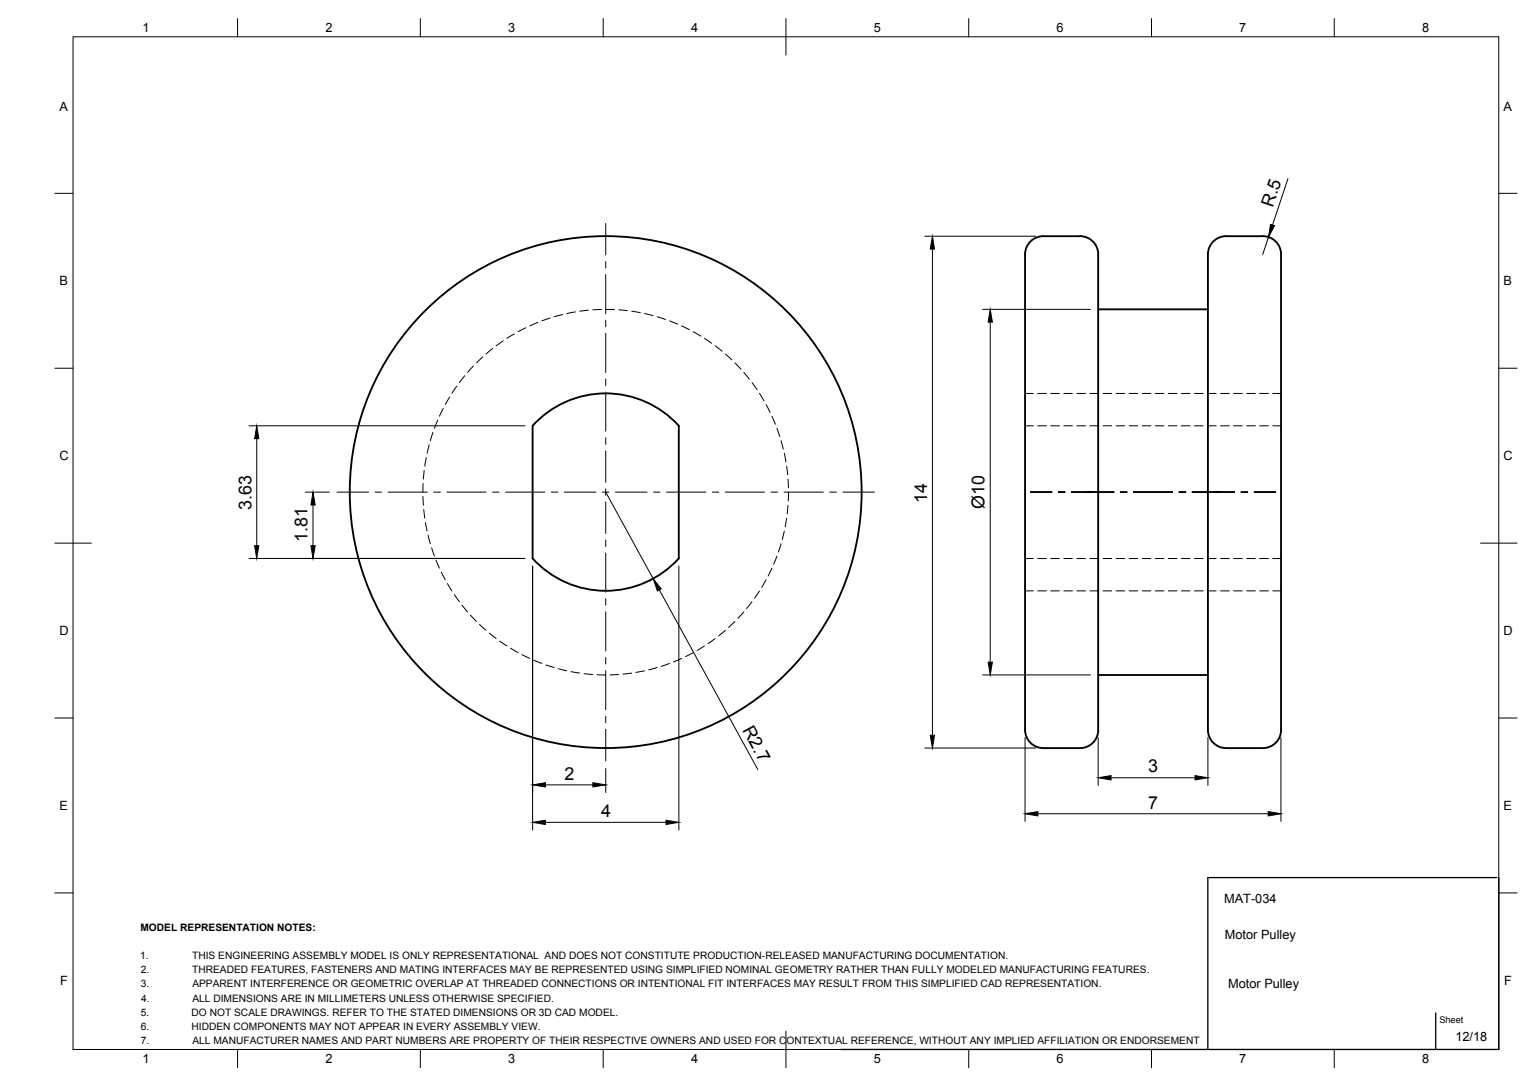
ISO-10303-21;
HEADER;
/* Generated by software containing ST-Developer
 * from STEP Tools, Inc. (www.steptools.com) 
 */

FILE_DESCRIPTION(
/* description */ ('STEP AP214'),
/* implementation_level */ '2;1');

FILE_NAME(
/* name */ 'Motor Pulley.step',
/* time_stamp */ '2026-11-14T09:24:36-08:00',
/* author */ (''),
/* organization */ (''),
/* preprocessor_version */ 'ST-DEVELOPER v20.2',
/* originating_system */ 'Autodesk Translation Framework v15.17.0.0',
/* authorisation */ '');

FILE_SCHEMA (('AUTOMOTIVE_DESIGN { 1 0 10303 214 3 1 1 }'));
ENDSEC;

DATA;
#10=MECHANICAL_DESIGN_GEOMETRIC_PRESENTATION_REPRESENTATION('',(#208),#18867);
#146=TOROIDAL_SURFACE('',#11512,6.5,0.5);
#147=TOROIDAL_SURFACE('',#11516,6.5,0.5);
#148=TOROIDAL_SURFACE('',#11521,6.5,0.5);
#149=TOROIDAL_SURFACE('',#11525,6.5,0.5);
#176=SHAPE_REPRESENTATION_RELATIONSHIP('SRR','None',#18940,#192);
#192=ADVANCED_BREP_SHAPE_REPRESENTATION('',(#232),#18856);
#208=STYLED_ITEM('',(#19027),#232);
#232=MANIFOLD_SOLID_BREP('Body1',#10963);
#319=FACE_BOUND('',#1599,.T.);
#320=FACE_BOUND('',#1601,.T.);
#321=FACE_BOUND('',#1603,.T.);
#322=FACE_BOUND('',#1605,.T.);
#513=PLANE('',#11535);
#514=PLANE('',#11536);
#515=PLANE('',#11537);
#516=PLANE('',#11540);
#517=PLANE('',#11543);
#518=PLANE('',#11545);
#927=FACE_OUTER_BOUND('',#1591,.T.);
#928=FACE_OUTER_BOUND('',#1592,.T.);
#929=FACE_OUTER_BOUND('',#1593,.T.);
#930=FACE_OUTER_BOUND('',#1594,.T.);
#931=FACE_OUTER_BOUND('',#1595,.T.);
#932=FACE_OUTER_BOUND('',#1596,.T.);
#933=FACE_OUTER_BOUND('',#1597,.T.);
#934=FACE_OUTER_BOUND('',#1598,.T.);
#935=FACE_OUTER_BOUND('',#1600,.T.);
#936=FACE_OUTER_BOUND('',#1602,.T.);
#937=FACE_OUTER_BOUND('',#1604,.T.);
#938=FACE_OUTER_BOUND('',#1606,.T.);
#939=FACE_OUTER_BOUND('',#1607,.T.);
#940=FACE_OUTER_BOUND('',#1608,.T.);
#941=FACE_OUTER_BOUND('',#1609,.T.);
#1591=EDGE_LOOP('',(#8120,#8121,#8122,#8123));
#1592=EDGE_LOOP('',(#8124,#8125,#8126,#8127,#8128));
#1593=EDGE_LOOP('',(#8129,#8130,#8131,#8132));
#1594=EDGE_LOOP('',(#8133,#8134,#8135,#8136,#8137));
#1595=EDGE_LOOP('',(#8138,#8139,#8140,#8141,#8142));
#1596=EDGE_LOOP('',(#8143,#8144,#8145,#8146));
#1597=EDGE_LOOP('',(#8147,#8148,#8149,#8150,#8151));
#1598=EDGE_LOOP('',(#8152));
#1599=EDGE_LOOP('',(#8153));
#1600=EDGE_LOOP('',(#8154));
#1601=EDGE_LOOP('',(#8155));
#1602=EDGE_LOOP('',(#8156));
#1603=EDGE_LOOP('',(#8157,#8158,#8159,#8160));
#1604=EDGE_LOOP('',(#8161));
#1605=EDGE_LOOP('',(#8162,#8163,#8164,#8165));
#1606=EDGE_LOOP('',(#8166,#8167,#8168,#8169));
#1607=EDGE_LOOP('',(#8170,#8171,#8172,#8173));
#1608=EDGE_LOOP('',(#8174,#8175,#8176,#8177));
#1609=EDGE_LOOP('',(#8178,#8179,#8180,#8181));
#2409=LINE('',#16685,#3423);
#2410=LINE('',#16690,#3424);
#2411=LINE('',#16693,#3425);
#2412=LINE('',#16701,#3426);
#2413=LINE('',#16704,#3427);
#2414=LINE('',#16710,#3428);
#2415=LINE('',#16713,#3429);
#2416=LINE('',#16715,#3430);
#2417=LINE('',#16716,#3431);
#2418=LINE('',#16718,#3432);
#2419=LINE('',#16720,#3433);
#3423=VECTOR('',#13409,7.);
#3424=VECTOR('',#13414,5.);
#3425=VECTOR('',#13419,7.);
#3426=VECTOR('',#13428,1000.);
#3427=VECTOR('',#13431,1000.);
#3428=VECTOR('',#13436,1000.);
#3429=VECTOR('',#13439,1000.);
#3430=VECTOR('',#13442,1000.);
#3431=VECTOR('',#13443,1000.);
#3432=VECTOR('',#13446,1000.);
#3433=VECTOR('',#13449,1000.);
#4215=CIRCLE('',#11513,7.);
#4216=CIRCLE('',#11514,0.5);
#4217=CIRCLE('',#11515,6.5);
#4218=CIRCLE('',#11517,7.);
#4219=CIRCLE('',#11518,7.);
#4220=CIRCLE('',#11519,0.5);
#4221=CIRCLE('',#11520,6.5);
#4222=CIRCLE('',#11522,7.);
#4223=CIRCLE('',#11523,0.5);
#4224=CIRCLE('',#11524,6.5);
#4225=CIRCLE('',#11526,7.);
#4226=CIRCLE('',#11527,7.);
#4227=CIRCLE('',#11528,0.5);
#4228=CIRCLE('',#11529,6.5);
#4229=CIRCLE('',#11532,5.);
#4230=CIRCLE('',#11533,5.);
#4231=CIRCLE('',#11538,2.7);
#4232=CIRCLE('',#11539,2.7);
#4233=CIRCLE('',#11541,2.7);
#4234=CIRCLE('',#11542,2.7);
#4910=VERTEX_POINT('',#16657);
#4911=VERTEX_POINT('',#16659);
#4912=VERTEX_POINT('',#16663);
#4913=VERTEX_POINT('',#16664);
#4914=VERTEX_POINT('',#16667);
#4915=VERTEX_POINT('',#16671);
#4916=VERTEX_POINT('',#16673);
#4917=VERTEX_POINT('',#16677);
#4918=VERTEX_POINT('',#16678);
#4919=VERTEX_POINT('',#16681);
#4920=VERTEX_POINT('',#16687);
#4921=VERTEX_POINT('',#16689);
#4922=VERTEX_POINT('',#16697);
#4923=VERTEX_POINT('',#16698);
#4924=VERTEX_POINT('',#16700);
#4925=VERTEX_POINT('',#16702);
#4926=VERTEX_POINT('',#16706);
#4927=VERTEX_POINT('',#16707);
#4928=VERTEX_POINT('',#16709);
#4929=VERTEX_POINT('',#16711);
#6093=EDGE_CURVE('',#4910,#4910,#4215,.T.);
#6094=EDGE_CURVE('',#4910,#4911,#4216,.T.);
#6095=EDGE_CURVE('',#4911,#4911,#4217,.T.);
#6096=EDGE_CURVE('',#4912,#4913,#4218,.T.);
#6097=EDGE_CURVE('',#4913,#4912,#4219,.T.);
#6098=EDGE_CURVE('',#4913,#4914,#4220,.T.);
#6099=EDGE_CURVE('',#4914,#4914,#4221,.T.);
#6100=EDGE_CURVE('',#4915,#4915,#4222,.T.);
#6101=EDGE_CURVE('',#4915,#4916,#4223,.T.);
#6102=EDGE_CURVE('',#4916,#4916,#4224,.T.);
#6103=EDGE_CURVE('',#4917,#4918,#4225,.T.);
#6104=EDGE_CURVE('',#4918,#4917,#4226,.T.);
#6105=EDGE_CURVE('',#4918,#4919,#4227,.T.);
#6106=EDGE_CURVE('',#4919,#4919,#4228,.T.);
#6107=EDGE_CURVE('',#4912,#4910,#2409,.T.);
#6108=EDGE_CURVE('',#4920,#4920,#4229,.T.);
#6109=EDGE_CURVE('',#4920,#4921,#2410,.T.);
#6110=EDGE_CURVE('',#4921,#4921,#4230,.T.);
#6111=EDGE_CURVE('',#4917,#4915,#2411,.T.);
#6112=EDGE_CURVE('',#4922,#4923,#4231,.T.);
#6113=EDGE_CURVE('',#4923,#4924,#2412,.T.);
#6114=EDGE_CURVE('',#4924,#4925,#4232,.T.);
#6115=EDGE_CURVE('',#4922,#4925,#2413,.T.);
#6116=EDGE_CURVE('',#4926,#4927,#4233,.T.);
#6117=EDGE_CURVE('',#4928,#4926,#2414,.T.);
#6118=EDGE_CURVE('',#4929,#4928,#4234,.T.);
#6119=EDGE_CURVE('',#4929,#4927,#2415,.T.);
#6120=EDGE_CURVE('',#4923,#4928,#2416,.T.);
#6121=EDGE_CURVE('',#4924,#4926,#2417,.T.);
#6122=EDGE_CURVE('',#4922,#4929,#2418,.T.);
#6123=EDGE_CURVE('',#4925,#4927,#2419,.T.);
#8120=ORIENTED_EDGE('',*,*,#6093,.F.);
#8121=ORIENTED_EDGE('',*,*,#6094,.T.);
#8122=ORIENTED_EDGE('',*,*,#6095,.F.);
#8123=ORIENTED_EDGE('',*,*,#6094,.F.);
#8124=ORIENTED_EDGE('',*,*,#6096,.F.);
#8125=ORIENTED_EDGE('',*,*,#6097,.F.);
#8126=ORIENTED_EDGE('',*,*,#6098,.T.);
#8127=ORIENTED_EDGE('',*,*,#6099,.F.);
#8128=ORIENTED_EDGE('',*,*,#6098,.F.);
#8129=ORIENTED_EDGE('',*,*,#6100,.F.);
#8130=ORIENTED_EDGE('',*,*,#6101,.T.);
#8131=ORIENTED_EDGE('',*,*,#6102,.F.);
#8132=ORIENTED_EDGE('',*,*,#6101,.F.);
#8133=ORIENTED_EDGE('',*,*,#6103,.F.);
#8134=ORIENTED_EDGE('',*,*,#6104,.F.);
#8135=ORIENTED_EDGE('',*,*,#6105,.T.);
#8136=ORIENTED_EDGE('',*,*,#6106,.F.);
#8137=ORIENTED_EDGE('',*,*,#6105,.F.);
#8138=ORIENTED_EDGE('',*,*,#6096,.T.);
#8139=ORIENTED_EDGE('',*,*,#6097,.T.);
#8140=ORIENTED_EDGE('',*,*,#6107,.T.);
#8141=ORIENTED_EDGE('',*,*,#6093,.T.);
#8142=ORIENTED_EDGE('',*,*,#6107,.F.);
#8143=ORIENTED_EDGE('',*,*,#6108,.F.);
#8144=ORIENTED_EDGE('',*,*,#6109,.T.);
#8145=ORIENTED_EDGE('',*,*,#6110,.T.);
#8146=ORIENTED_EDGE('',*,*,#6109,.F.);
#8147=ORIENTED_EDGE('',*,*,#6103,.T.);
#8148=ORIENTED_EDGE('',*,*,#6104,.T.);
#8149=ORIENTED_EDGE('',*,*,#6111,.T.);
#8150=ORIENTED_EDGE('',*,*,#6100,.T.);
#8151=ORIENTED_EDGE('',*,*,#6111,.F.);
#8152=ORIENTED_EDGE('',*,*,#6102,.T.);
#8153=ORIENTED_EDGE('',*,*,#6108,.T.);
#8154=ORIENTED_EDGE('',*,*,#6099,.T.);
#8155=ORIENTED_EDGE('',*,*,#6110,.F.);
#8156=ORIENTED_EDGE('',*,*,#6095,.T.);
#8157=ORIENTED_EDGE('',*,*,#6112,.T.);
#8158=ORIENTED_EDGE('',*,*,#6113,.T.);
#8159=ORIENTED_EDGE('',*,*,#6114,.T.);
#8160=ORIENTED_EDGE('',*,*,#6115,.F.);
#8161=ORIENTED_EDGE('',*,*,#6106,.T.);
#8162=ORIENTED_EDGE('',*,*,#6116,.F.);
#8163=ORIENTED_EDGE('',*,*,#6117,.F.);
#8164=ORIENTED_EDGE('',*,*,#6118,.F.);
#8165=ORIENTED_EDGE('',*,*,#6119,.T.);
#8166=ORIENTED_EDGE('',*,*,#6120,.T.);
#8167=ORIENTED_EDGE('',*,*,#6117,.T.);
#8168=ORIENTED_EDGE('',*,*,#6121,.F.);
#8169=ORIENTED_EDGE('',*,*,#6113,.F.);
#8170=ORIENTED_EDGE('',*,*,#6122,.T.);
#8171=ORIENTED_EDGE('',*,*,#6118,.T.);
#8172=ORIENTED_EDGE('',*,*,#6120,.F.);
#8173=ORIENTED_EDGE('',*,*,#6112,.F.);
#8174=ORIENTED_EDGE('',*,*,#6115,.T.);
#8175=ORIENTED_EDGE('',*,*,#6123,.T.);
#8176=ORIENTED_EDGE('',*,*,#6119,.F.);
#8177=ORIENTED_EDGE('',*,*,#6122,.F.);
#8178=ORIENTED_EDGE('',*,*,#6121,.T.);
#8179=ORIENTED_EDGE('',*,*,#6116,.T.);
#8180=ORIENTED_EDGE('',*,*,#6123,.F.);
#8181=ORIENTED_EDGE('',*,*,#6114,.F.);
#10220=CYLINDRICAL_SURFACE('',#11530,7.);
#10221=CYLINDRICAL_SURFACE('',#11531,5.);
#10222=CYLINDRICAL_SURFACE('',#11534,7.);
#10223=CYLINDRICAL_SURFACE('',#11544,2.7);
#10224=CYLINDRICAL_SURFACE('',#11546,2.7);
#10564=ADVANCED_FACE('',(#927),#146,.T.);
#10565=ADVANCED_FACE('',(#928),#147,.T.);
#10566=ADVANCED_FACE('',(#929),#148,.T.);
#10567=ADVANCED_FACE('',(#930),#149,.T.);
#10568=ADVANCED_FACE('',(#931),#10220,.T.);
#10569=ADVANCED_FACE('',(#932),#10221,.T.);
#10570=ADVANCED_FACE('',(#933),#10222,.T.);
#10571=ADVANCED_FACE('',(#934,#319),#513,.F.);
#10572=ADVANCED_FACE('',(#935,#320),#514,.F.);
#10573=ADVANCED_FACE('',(#936,#321),#515,.F.);
#10574=ADVANCED_FACE('',(#937,#322),#516,.F.);
#10575=ADVANCED_FACE('',(#938),#517,.F.);
#10576=ADVANCED_FACE('',(#939),#10223,.F.);
#10577=ADVANCED_FACE('',(#940),#518,.T.);
#10578=ADVANCED_FACE('',(#941),#10224,.F.);
#10963=CLOSED_SHELL('',(#10564,#10565,#10566,#10567,#10568,#10569,#10570,
#10571,#10572,#10573,#10574,#10575,#10576,#10577,#10578));
#11511=AXIS2_PLACEMENT_3D('',#16655,#13369,#13370);
#11512=AXIS2_PLACEMENT_3D('',#16656,#13371,#13372);
#11513=AXIS2_PLACEMENT_3D('',#16658,#13373,#13374);
#11514=AXIS2_PLACEMENT_3D('',#16660,#13375,#13376);
#11515=AXIS2_PLACEMENT_3D('',#16661,#13377,#13378);
#11516=AXIS2_PLACEMENT_3D('',#16662,#13379,#13380);
#11517=AXIS2_PLACEMENT_3D('',#16665,#13381,#13382);
#11518=AXIS2_PLACEMENT_3D('',#16666,#13383,#13384);
#11519=AXIS2_PLACEMENT_3D('',#16668,#13385,#13386);
#11520=AXIS2_PLACEMENT_3D('',#16669,#13387,#13388);
#11521=AXIS2_PLACEMENT_3D('',#16670,#13389,#13390);
#11522=AXIS2_PLACEMENT_3D('',#16672,#13391,#13392);
#11523=AXIS2_PLACEMENT_3D('',#16674,#13393,#13394);
#11524=AXIS2_PLACEMENT_3D('',#16675,#13395,#13396);
#11525=AXIS2_PLACEMENT_3D('',#16676,#13397,#13398);
#11526=AXIS2_PLACEMENT_3D('',#16679,#13399,#13400);
#11527=AXIS2_PLACEMENT_3D('',#16680,#13401,#13402);
#11528=AXIS2_PLACEMENT_3D('',#16682,#13403,#13404);
#11529=AXIS2_PLACEMENT_3D('',#16683,#13405,#13406);
#11530=AXIS2_PLACEMENT_3D('',#16684,#13407,#13408);
#11531=AXIS2_PLACEMENT_3D('',#16686,#13410,#13411);
#11532=AXIS2_PLACEMENT_3D('',#16688,#13412,#13413);
#11533=AXIS2_PLACEMENT_3D('',#16691,#13415,#13416);
#11534=AXIS2_PLACEMENT_3D('',#16692,#13417,#13418);
#11535=AXIS2_PLACEMENT_3D('',#16694,#13420,#13421);
#11536=AXIS2_PLACEMENT_3D('',#16695,#13422,#13423);
#11537=AXIS2_PLACEMENT_3D('',#16696,#13424,#13425);
#11538=AXIS2_PLACEMENT_3D('',#16699,#13426,#13427);
#11539=AXIS2_PLACEMENT_3D('',#16703,#13429,#13430);
#11540=AXIS2_PLACEMENT_3D('',#16705,#13432,#13433);
#11541=AXIS2_PLACEMENT_3D('',#16708,#13434,#13435);
#11542=AXIS2_PLACEMENT_3D('',#16712,#13437,#13438);
#11543=AXIS2_PLACEMENT_3D('',#16714,#13440,#13441);
#11544=AXIS2_PLACEMENT_3D('',#16717,#13444,#13445);
#11545=AXIS2_PLACEMENT_3D('',#16719,#13447,#13448);
#11546=AXIS2_PLACEMENT_3D('',#16721,#13450,#13451);
#13369=DIRECTION('axis',(0.,0.,1.));
#13370=DIRECTION('refdir',(1.,0.,0.));
#13371=DIRECTION('center_axis',(-1.,0.,0.));
#13372=DIRECTION('ref_axis',(0.,0.,1.));
#13373=DIRECTION('center_axis',(-1.,0.,0.));
#13374=DIRECTION('ref_axis',(0.,0.,1.));
#13375=DIRECTION('center_axis',(0.,-1.,1.22464679914735E-16));
#13376=DIRECTION('ref_axis',(0.,-1.22464679914735E-16,-1.));
#13377=DIRECTION('center_axis',(1.,0.,0.));
#13378=DIRECTION('ref_axis',(0.,0.,1.));
#13379=DIRECTION('center_axis',(1.,0.,0.));
#13380=DIRECTION('ref_axis',(0.,0.,-1.));
#13381=DIRECTION('center_axis',(1.,0.,0.));
#13382=DIRECTION('ref_axis',(0.,0.,-1.));
#13383=DIRECTION('center_axis',(1.,0.,0.));
#13384=DIRECTION('ref_axis',(0.,0.,-1.));
#13385=DIRECTION('center_axis',(0.,-1.,-1.22464679914735E-16));
#13386=DIRECTION('ref_axis',(0.,-1.22464679914735E-16,1.));
#13387=DIRECTION('center_axis',(-1.,0.,0.));
#13388=DIRECTION('ref_axis',(0.,0.,-1.));
#13389=DIRECTION('center_axis',(-1.,0.,0.));
#13390=DIRECTION('ref_axis',(0.,0.,1.));
#13391=DIRECTION('center_axis',(-1.,0.,0.));
#13392=DIRECTION('ref_axis',(0.,0.,1.));
#13393=DIRECTION('center_axis',(0.,-1.,1.22464679914735E-16));
#13394=DIRECTION('ref_axis',(0.,-1.22464679914735E-16,-1.));
#13395=DIRECTION('center_axis',(1.,0.,0.));
#13396=DIRECTION('ref_axis',(0.,0.,1.));
#13397=DIRECTION('center_axis',(1.,0.,0.));
#13398=DIRECTION('ref_axis',(0.,0.,-1.));
#13399=DIRECTION('center_axis',(1.,0.,0.));
#13400=DIRECTION('ref_axis',(0.,0.,-1.));
#13401=DIRECTION('center_axis',(1.,0.,0.));
#13402=DIRECTION('ref_axis',(0.,0.,-1.));
#13403=DIRECTION('center_axis',(0.,-1.,-1.22464679914735E-16));
#13404=DIRECTION('ref_axis',(0.,-1.22464679914735E-16,1.));
#13405=DIRECTION('center_axis',(-1.,0.,0.));
#13406=DIRECTION('ref_axis',(0.,0.,-1.));
#13407=DIRECTION('center_axis',(-1.,0.,0.));
#13408=DIRECTION('ref_axis',(0.,0.,1.));
#13409=DIRECTION('',(1.,0.,0.));
#13410=DIRECTION('center_axis',(-1.,0.,0.));
#13411=DIRECTION('ref_axis',(0.,0.,1.));
#13412=DIRECTION('center_axis',(-1.,0.,0.));
#13413=DIRECTION('ref_axis',(0.,0.,1.));
#13414=DIRECTION('',(1.,0.,0.));
#13415=DIRECTION('center_axis',(-1.,0.,0.));
#13416=DIRECTION('ref_axis',(0.,0.,1.));
#13417=DIRECTION('center_axis',(-1.,0.,0.));
#13418=DIRECTION('ref_axis',(0.,0.,1.));
#13419=DIRECTION('',(1.,0.,0.));
#13420=DIRECTION('center_axis',(-1.,0.,0.));
#13421=DIRECTION('ref_axis',(0.,0.,1.));
#13422=DIRECTION('center_axis',(1.,0.,0.));
#13423=DIRECTION('ref_axis',(0.,0.,-1.));
#13424=DIRECTION('center_axis',(-1.,0.,0.));
#13425=DIRECTION('ref_axis',(0.,0.,1.));
#13426=DIRECTION('center_axis',(-1.,0.,0.));
#13427=DIRECTION('ref_axis',(0.,0.,1.));
#13428=DIRECTION('',(0.,1.,0.));
#13429=DIRECTION('center_axis',(-1.,0.,0.));
#13430=DIRECTION('ref_axis',(0.,0.,1.));
#13431=DIRECTION('',(0.,1.,-4.7819200545485E-16));
#13432=DIRECTION('center_axis',(1.,0.,0.));
#13433=DIRECTION('ref_axis',(0.,0.,-1.));
#13434=DIRECTION('center_axis',(-1.,0.,0.));
#13435=DIRECTION('ref_axis',(0.,0.,1.));
#13436=DIRECTION('',(0.,1.,0.));
#13437=DIRECTION('center_axis',(-1.,0.,0.));
#13438=DIRECTION('ref_axis',(0.,0.,1.));
#13439=DIRECTION('',(0.,1.,-4.7819200545485E-16));
#13440=DIRECTION('center_axis',(0.,0.,1.));
#13441=DIRECTION('ref_axis',(1.,0.,0.));
#13442=DIRECTION('',(-1.,0.,0.));
#13443=DIRECTION('',(-1.,0.,0.));
#13444=DIRECTION('center_axis',(-1.,0.,0.));
#13445=DIRECTION('ref_axis',(0.,0.,1.));
#13446=DIRECTION('',(-1.,0.,0.));
#13447=DIRECTION('center_axis',(0.,4.7819200545485E-16,1.));
#13448=DIRECTION('ref_axis',(0.,-1.,4.7819200545485E-16));
#13449=DIRECTION('',(-1.,0.,0.));
#13450=DIRECTION('center_axis',(-1.,0.,0.));
#13451=DIRECTION('ref_axis',(0.,0.,1.));
#16655=CARTESIAN_POINT('',(0.,0.,0.));
#16656=CARTESIAN_POINT('Origin',(3.,0.,0.));
#16657=CARTESIAN_POINT('',(3.,-8.57252759403147E-16,-7.));
#16658=CARTESIAN_POINT('Origin',(3.,0.,0.));
#16659=CARTESIAN_POINT('',(3.5,-7.9602041944578E-16,-6.5));
#16660=CARTESIAN_POINT('Origin',(3.,-7.9602041944578E-16,-6.5));
#16661=CARTESIAN_POINT('Origin',(3.5,0.,0.));
#16662=CARTESIAN_POINT('Origin',(2.,0.,0.));
#16663=CARTESIAN_POINT('',(2.,8.57252759403147E-16,-7.));
#16664=CARTESIAN_POINT('',(2.,-8.57252759403147E-16,7.));
#16665=CARTESIAN_POINT('Origin',(2.,0.,0.));
#16666=CARTESIAN_POINT('Origin',(2.,0.,0.));
#16667=CARTESIAN_POINT('',(1.5,-7.9602041944578E-16,6.5));
#16668=CARTESIAN_POINT('Origin',(2.,-7.9602041944578E-16,6.5));
#16669=CARTESIAN_POINT('Origin',(1.5,0.,0.));
#16670=CARTESIAN_POINT('Origin',(-2.,0.,0.));
#16671=CARTESIAN_POINT('',(-2.,-8.57252759403147E-16,-7.));
#16672=CARTESIAN_POINT('Origin',(-2.,0.,0.));
#16673=CARTESIAN_POINT('',(-1.5,-7.9602041944578E-16,-6.5));
#16674=CARTESIAN_POINT('Origin',(-2.,-7.9602041944578E-16,-6.5));
#16675=CARTESIAN_POINT('Origin',(-1.5,0.,0.));
#16676=CARTESIAN_POINT('Origin',(-3.,0.,0.));
#16677=CARTESIAN_POINT('',(-3.,8.57252759403147E-16,-7.));
#16678=CARTESIAN_POINT('',(-3.,-8.57252759403147E-16,7.));
#16679=CARTESIAN_POINT('Origin',(-3.,0.,0.));
#16680=CARTESIAN_POINT('Origin',(-3.,0.,0.));
#16681=CARTESIAN_POINT('',(-3.5,-7.9602041944578E-16,6.5));
#16682=CARTESIAN_POINT('Origin',(-3.,-7.9602041944578E-16,6.5));
#16683=CARTESIAN_POINT('Origin',(-3.5,0.,0.));
#16684=CARTESIAN_POINT('Origin',(-3.5,0.,0.));
#16685=CARTESIAN_POINT('',(-3.5,-8.57252759403147E-16,-7.));
#16686=CARTESIAN_POINT('Origin',(-3.5,0.,0.));
#16687=CARTESIAN_POINT('',(-1.5,-6.12323399573677E-16,-5.));
#16688=CARTESIAN_POINT('Origin',(-1.5,0.,0.));
#16689=CARTESIAN_POINT('',(1.5,-6.12323399573677E-16,-5.));
#16690=CARTESIAN_POINT('',(-3.5,-6.12323399573677E-16,-5.));
#16691=CARTESIAN_POINT('Origin',(1.5,0.,0.));
#16692=CARTESIAN_POINT('Origin',(-3.5,0.,0.));
#16693=CARTESIAN_POINT('',(-3.5,-8.57252759403147E-16,-7.));
#16694=CARTESIAN_POINT('Origin',(-1.5,7.,0.));
#16695=CARTESIAN_POINT('Origin',(1.5,5.,0.));
#16696=CARTESIAN_POINT('Origin',(3.5,7.,0.));
#16697=CARTESIAN_POINT('',(3.5,-1.81383571472171,-2.));
#16698=CARTESIAN_POINT('',(3.5,-1.81383571472171,2.));
#16699=CARTESIAN_POINT('Origin',(3.5,0.,0.));
#16700=CARTESIAN_POINT('',(3.5,1.81383571472171,2.));
#16701=CARTESIAN_POINT('',(3.5,7.,2.));
#16702=CARTESIAN_POINT('',(3.5,1.81383571472171,-2.));
#16703=CARTESIAN_POINT('Origin',(3.5,0.,0.));
#16704=CARTESIAN_POINT('',(3.5,7.,-2.));
#16705=CARTESIAN_POINT('Origin',(-3.5,0.,0.));
#16706=CARTESIAN_POINT('',(-3.5,1.81383571472171,2.));
#16707=CARTESIAN_POINT('',(-3.5,1.81383571472171,-2.));
#16708=CARTESIAN_POINT('Origin',(-3.5,0.,0.));
#16709=CARTESIAN_POINT('',(-3.5,-1.81383571472171,2.));
#16710=CARTESIAN_POINT('',(-3.5,0.,2.));
#16711=CARTESIAN_POINT('',(-3.5,-1.81383571472171,-2.));
#16712=CARTESIAN_POINT('Origin',(-3.5,0.,0.));
#16713=CARTESIAN_POINT('',(-3.5,-9.563840109097E-16,-2.));
#16714=CARTESIAN_POINT('Origin',(6.5,0.,2.));
#16715=CARTESIAN_POINT('',(6.5,-1.81383571472171,2.));
#16716=CARTESIAN_POINT('',(6.5,1.81383571472171,2.));
#16717=CARTESIAN_POINT('Origin',(6.5,0.,0.));
#16718=CARTESIAN_POINT('',(6.5,-1.81383571472171,-2.));
#16719=CARTESIAN_POINT('Origin',(6.5,-9.563840109097E-16,-2.));
#16720=CARTESIAN_POINT('',(6.5,1.81383571472171,-2.));
#16721=CARTESIAN_POINT('Origin',(6.5,0.,0.));
#18838=UNCERTAINTY_MEASURE_WITH_UNIT(LENGTH_MEASURE(0.01),#18868,
'DISTANCE_ACCURACY_VALUE',
'Maximum model space distance between geometric entities at asserted c
onnectivities');
#18849=UNCERTAINTY_MEASURE_WITH_UNIT(LENGTH_MEASURE(0.01),#18868,
'DISTANCE_ACCURACY_VALUE',
'Maximum model space distance between geometric entities at asserted c
onnectivities');
#18856=(
GEOMETRIC_REPRESENTATION_CONTEXT(3)
GLOBAL_UNCERTAINTY_ASSIGNED_CONTEXT((#18838))
GLOBAL_UNIT_ASSIGNED_CONTEXT((#18868,#18870,#18871))
REPRESENTATION_CONTEXT('','3D')
);
#18867=(
GEOMETRIC_REPRESENTATION_CONTEXT(3)
GLOBAL_UNCERTAINTY_ASSIGNED_CONTEXT((#18849))
GLOBAL_UNIT_ASSIGNED_CONTEXT((#18868,#18870,#18871))
REPRESENTATION_CONTEXT('','3D')
);
#18868=(
LENGTH_UNIT()
NAMED_UNIT(*)
SI_UNIT(.MILLI.,.METRE.)
);
#18870=(
NAMED_UNIT(*)
PLANE_ANGLE_UNIT()
SI_UNIT($,.RADIAN.)
);
#18871=(
NAMED_UNIT(*)
SI_UNIT($,.STERADIAN.)
SOLID_ANGLE_UNIT()
);
#18878=SHAPE_DEFINITION_REPRESENTATION(#18895,#18940);
#18895=PRODUCT_DEFINITION_SHAPE('',$,#18958);
#18940=SHAPE_REPRESENTATION('',(#11511),#18856);
#18951=PRODUCT_DEFINITION_CONTEXT('part definition',#19004,'design');
#18958=PRODUCT_DEFINITION('Motor Pulley','Motor Pulley',#18975,#18951);
#18975=PRODUCT_DEFINITION_FORMATION('',$,#19012);
#19004=APPLICATION_CONTEXT(
'Core Data for Automotive Mechanical Design Process');
#19005=PRODUCT_CONTEXT('part definition',#19004,'mechanical');
#19012=PRODUCT('Motor Pulley','Motor Pulley',$,(#19005));
#19027=PRESENTATION_STYLE_ASSIGNMENT((#19033));
#19033=SURFACE_STYLE_USAGE(.BOTH.,#19039);
#19039=SURFACE_SIDE_STYLE('',(#19045));
#19045=SURFACE_STYLE_FILL_AREA(#19051);
#19051=FILL_AREA_STYLE('Opaque(122,133,145)',(#19057));
#19057=FILL_AREA_STYLE_COLOUR('Opaque(122,133,145)',#19063);
#19063=COLOUR_RGB('Opaque(122,133,145)',0.47843137254902,0.52156862745098,
0.568627450980392);
ENDSEC;
END-ISO-10303-21;
